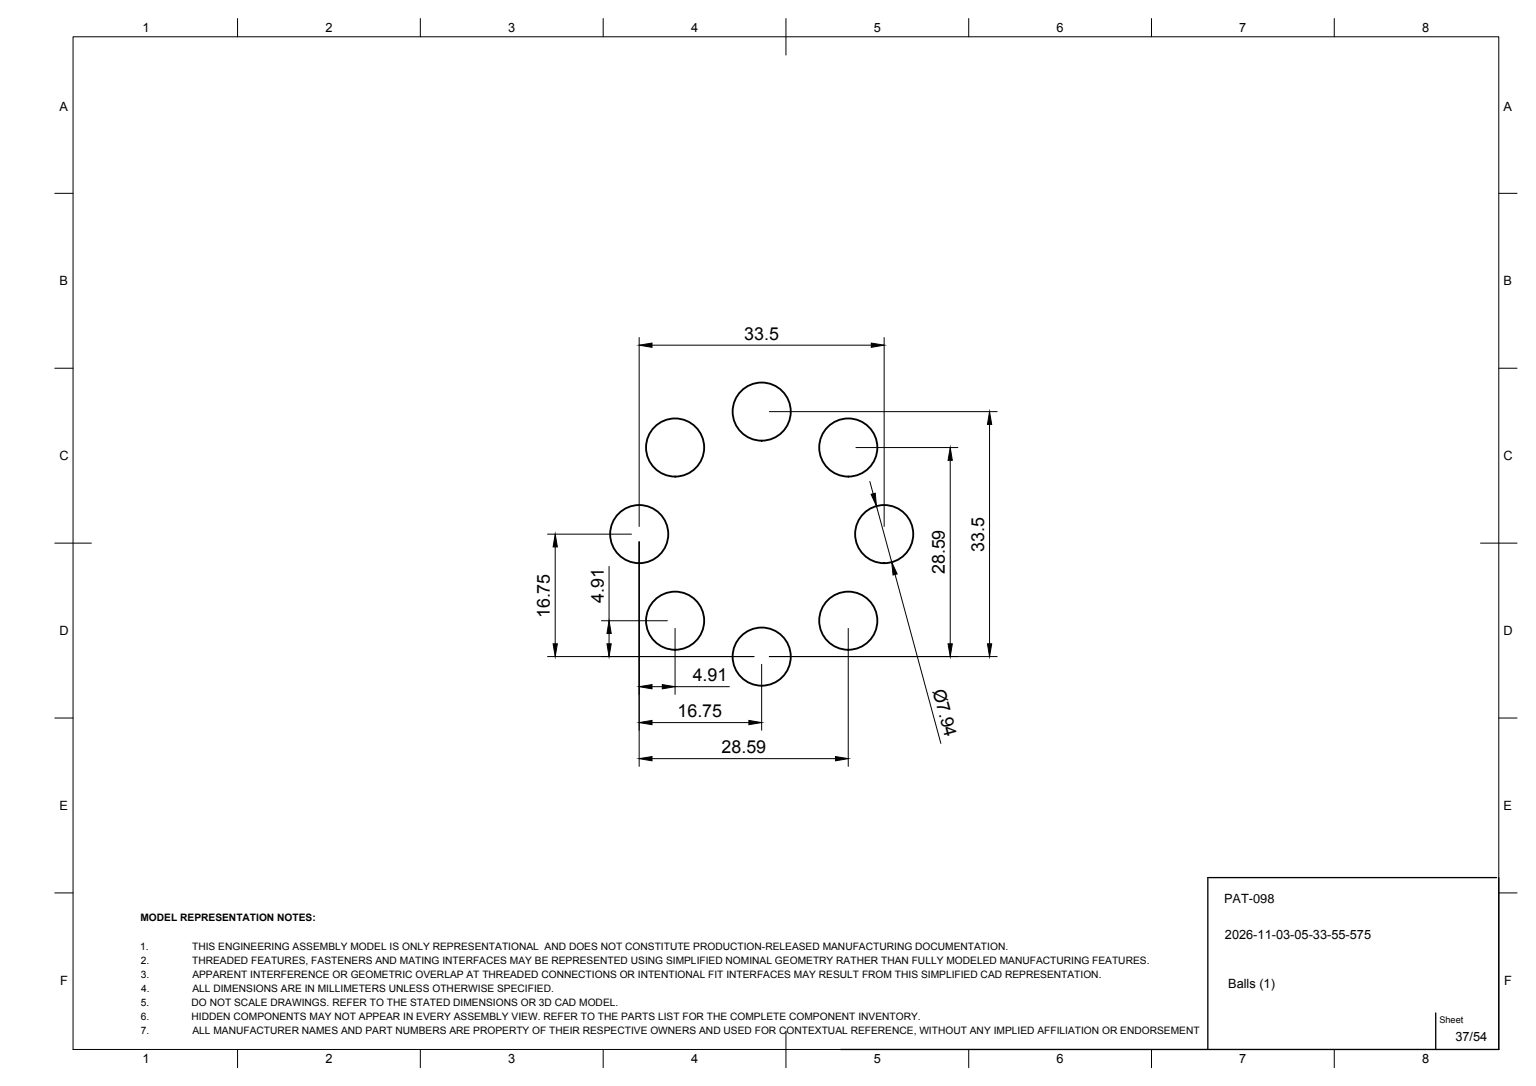
ISO-10303-21;
HEADER;
/* Generated by software containing ST-Developer
 * from STEP Tools, Inc. (www.steptools.com) 
 */

FILE_DESCRIPTION(
/* description */ ('Spring compression tester'),
/* implementation_level */ '2;1');

FILE_NAME(
/* name */ 'Balls (1).step',
/* time_stamp */ '2026-10-28T03:24:11-07:00',
/* author */ (''),
/* organization */ (''),
/* preprocessor_version */ 'ST-DEVELOPER v20.2',
/* originating_system */ 'Autodesk Translation Framework v15.17.0.0',
/* authorisation */ '');

FILE_SCHEMA (('AUTOMOTIVE_DESIGN { 1 0 10303 214 3 1 1 }'));
ENDSEC;

DATA;
#10=MECHANICAL_DESIGN_GEOMETRIC_PRESENTATION_REPRESENTATION('',(#1141,#1142,#1143,#1144,#1145,#1146,#1147,#1148),#43521);
#911=SPHERICAL_SURFACE('',#20162,0.3969);
#912=SPHERICAL_SURFACE('',#20164,0.3969);
#913=SPHERICAL_SURFACE('',#20166,0.3969);
#914=SPHERICAL_SURFACE('',#20168,0.3969);
#915=SPHERICAL_SURFACE('',#20170,0.3969);
#916=SPHERICAL_SURFACE('',#20172,0.3969);
#917=SPHERICAL_SURFACE('',#20174,0.3969);
#918=SPHERICAL_SURFACE('',#20176,0.3969);
#1014=SHAPE_REPRESENTATION_RELATIONSHIP('SRR','None',#43828,#1074);
#1074=ADVANCED_BREP_SHAPE_REPRESENTATION('',(#1215,#1216,#1217,#1218,#1219,
#1220,#1221,#1222),#43488);
#1141=STYLED_ITEM('',(#44202),#1215);
#1142=STYLED_ITEM('',(#44202),#1216);
#1143=STYLED_ITEM('',(#44202),#1217);
#1144=STYLED_ITEM('',(#44202),#1218);
#1145=STYLED_ITEM('',(#44202),#1219);
#1146=STYLED_ITEM('',(#44202),#1220);
#1147=STYLED_ITEM('',(#44202),#1221);
#1148=STYLED_ITEM('',(#44202),#1222);
#1215=MANIFOLD_SOLID_BREP('Body1',#18579);
#1216=MANIFOLD_SOLID_BREP('Body2',#18580);
#1217=MANIFOLD_SOLID_BREP('Body3',#18581);
#1218=MANIFOLD_SOLID_BREP('Body4',#18582);
#1219=MANIFOLD_SOLID_BREP('Body5',#18583);
#1220=MANIFOLD_SOLID_BREP('Body6',#18584);
#1221=MANIFOLD_SOLID_BREP('Body7',#18585);
#1222=MANIFOLD_SOLID_BREP('Body8',#18586);
#2660=FACE_OUTER_BOUND('',#3923,.T.);
#2661=FACE_OUTER_BOUND('',#3924,.T.);
#2662=FACE_OUTER_BOUND('',#3925,.T.);
#2663=FACE_OUTER_BOUND('',#3926,.T.);
#2664=FACE_OUTER_BOUND('',#3927,.T.);
#2665=FACE_OUTER_BOUND('',#3928,.T.);
#2666=FACE_OUTER_BOUND('',#3929,.T.);
#2667=FACE_OUTER_BOUND('',#3930,.T.);
#3923=EDGE_LOOP('',(#14383,#14384));
#3924=EDGE_LOOP('',(#14385,#14386));
#3925=EDGE_LOOP('',(#14387,#14388));
#3926=EDGE_LOOP('',(#14389,#14390));
#3927=EDGE_LOOP('',(#14391,#14392));
#3928=EDGE_LOOP('',(#14393,#14394));
#3929=EDGE_LOOP('',(#14395,#14396));
#3930=EDGE_LOOP('',(#14397,#14398));
#7818=CIRCLE('',#20163,0.3969);
#7819=CIRCLE('',#20165,0.3969);
#7820=CIRCLE('',#20167,0.3969);
#7821=CIRCLE('',#20169,0.3969);
#7822=CIRCLE('',#20171,0.3969);
#7823=CIRCLE('',#20173,0.3969);
#7824=CIRCLE('',#20175,0.3969);
#7825=CIRCLE('',#20177,0.3969);
#8863=VERTEX_POINT('',#29087);
#8864=VERTEX_POINT('',#29088);
#8865=VERTEX_POINT('',#29091);
#8866=VERTEX_POINT('',#29092);
#8867=VERTEX_POINT('',#29095);
#8868=VERTEX_POINT('',#29096);
#8869=VERTEX_POINT('',#29099);
#8870=VERTEX_POINT('',#29100);
#8871=VERTEX_POINT('',#29103);
#8872=VERTEX_POINT('',#29104);
#8873=VERTEX_POINT('',#29107);
#8874=VERTEX_POINT('',#29108);
#8875=VERTEX_POINT('',#29111);
#8876=VERTEX_POINT('',#29112);
#8877=VERTEX_POINT('',#29115);
#8878=VERTEX_POINT('',#29116);
#10856=EDGE_CURVE('',#8863,#8864,#7818,.T.);
#10857=EDGE_CURVE('',#8865,#8866,#7819,.T.);
#10858=EDGE_CURVE('',#8867,#8868,#7820,.T.);
#10859=EDGE_CURVE('',#8869,#8870,#7821,.T.);
#10860=EDGE_CURVE('',#8871,#8872,#7822,.T.);
#10861=EDGE_CURVE('',#8873,#8874,#7823,.T.);
#10862=EDGE_CURVE('',#8875,#8876,#7824,.T.);
#10863=EDGE_CURVE('',#8877,#8878,#7825,.T.);
#14383=ORIENTED_EDGE('',*,*,#10856,.T.);
#14384=ORIENTED_EDGE('',*,*,#10856,.F.);
#14385=ORIENTED_EDGE('',*,*,#10857,.T.);
#14386=ORIENTED_EDGE('',*,*,#10857,.F.);
#14387=ORIENTED_EDGE('',*,*,#10858,.T.);
#14388=ORIENTED_EDGE('',*,*,#10858,.F.);
#14389=ORIENTED_EDGE('',*,*,#10859,.T.);
#14390=ORIENTED_EDGE('',*,*,#10859,.F.);
#14391=ORIENTED_EDGE('',*,*,#10860,.T.);
#14392=ORIENTED_EDGE('',*,*,#10860,.F.);
#14393=ORIENTED_EDGE('',*,*,#10861,.T.);
#14394=ORIENTED_EDGE('',*,*,#10861,.F.);
#14395=ORIENTED_EDGE('',*,*,#10862,.T.);
#14396=ORIENTED_EDGE('',*,*,#10862,.F.);
#14397=ORIENTED_EDGE('',*,*,#10863,.T.);
#14398=ORIENTED_EDGE('',*,*,#10863,.F.);
#17984=ADVANCED_FACE('',(#2660),#911,.T.);
#17985=ADVANCED_FACE('',(#2661),#912,.T.);
#17986=ADVANCED_FACE('',(#2662),#913,.T.);
#17987=ADVANCED_FACE('',(#2663),#914,.T.);
#17988=ADVANCED_FACE('',(#2664),#915,.T.);
#17989=ADVANCED_FACE('',(#2665),#916,.T.);
#17990=ADVANCED_FACE('',(#2666),#917,.T.);
#17991=ADVANCED_FACE('',(#2667),#918,.T.);
#18579=CLOSED_SHELL('',(#17984));
#18580=CLOSED_SHELL('',(#17985));
#18581=CLOSED_SHELL('',(#17986));
#18582=CLOSED_SHELL('',(#17987));
#18583=CLOSED_SHELL('',(#17988));
#18584=CLOSED_SHELL('',(#17989));
#18585=CLOSED_SHELL('',(#17990));
#18586=CLOSED_SHELL('',(#17991));
#20161=AXIS2_PLACEMENT_3D('',#29085,#23671,#23672);
#20162=AXIS2_PLACEMENT_3D('',#29086,#23673,#23674);
#20163=AXIS2_PLACEMENT_3D('',#29089,#23675,#23676);
#20164=AXIS2_PLACEMENT_3D('',#29090,#23677,#23678);
#20165=AXIS2_PLACEMENT_3D('',#29093,#23679,#23680);
#20166=AXIS2_PLACEMENT_3D('',#29094,#23681,#23682);
#20167=AXIS2_PLACEMENT_3D('',#29097,#23683,#23684);
#20168=AXIS2_PLACEMENT_3D('',#29098,#23685,#23686);
#20169=AXIS2_PLACEMENT_3D('',#29101,#23687,#23688);
#20170=AXIS2_PLACEMENT_3D('',#29102,#23689,#23690);
#20171=AXIS2_PLACEMENT_3D('',#29105,#23691,#23692);
#20172=AXIS2_PLACEMENT_3D('',#29106,#23693,#23694);
#20173=AXIS2_PLACEMENT_3D('',#29109,#23695,#23696);
#20174=AXIS2_PLACEMENT_3D('',#29110,#23697,#23698);
#20175=AXIS2_PLACEMENT_3D('',#29113,#23699,#23700);
#20176=AXIS2_PLACEMENT_3D('',#29114,#23701,#23702);
#20177=AXIS2_PLACEMENT_3D('',#29117,#23703,#23704);
#23671=DIRECTION('axis',(0.,0.,1.));
#23672=DIRECTION('refdir',(1.,0.,0.));
#23673=DIRECTION('center_axis',(0.,0.,1.));
#23674=DIRECTION('ref_axis',(1.,0.,0.));
#23675=DIRECTION('center_axis',(1.22464679914735E-16,-1.,0.));
#23676=DIRECTION('ref_axis',(-1.,-1.22464679914735E-16,0.));
#23677=DIRECTION('center_axis',(0.707106781186548,0.,0.707106781186548));
#23678=DIRECTION('ref_axis',(0.707106781186548,0.,-0.707106781186548));
#23679=DIRECTION('center_axis',(8.65956056235493E-17,-1.,-8.65956056235493E-17));
#23680=DIRECTION('ref_axis',(-0.707106781186548,-1.22464679914735E-16,0.707106781186548));
#23681=DIRECTION('center_axis',(1.,0.,0.));
#23682=DIRECTION('ref_axis',(6.12323399573677E-17,0.,-1.));
#23683=DIRECTION('center_axis',(7.49879891330929E-33,-1.,-1.22464679914735E-16));
#23684=DIRECTION('ref_axis',(-6.12323399573677E-17,-1.22464679914735E-16,
1.));
#23685=DIRECTION('center_axis',(0.707106781186548,0.,-0.707106781186548));
#23686=DIRECTION('ref_axis',(-0.707106781186548,0.,-0.707106781186548));
#23687=DIRECTION('center_axis',(-8.65956056235493E-17,-1.,-8.65956056235493E-17));
#23688=DIRECTION('ref_axis',(0.707106781186548,-1.22464679914735E-16,0.707106781186548));
#23689=DIRECTION('center_axis',(0.,0.,-1.));
#23690=DIRECTION('ref_axis',(-1.,0.,-1.22464679914735E-16));
#23691=DIRECTION('center_axis',(-1.22464679914735E-16,-1.,-1.49975978266186E-32));
#23692=DIRECTION('ref_axis',(1.,-1.22464679914735E-16,1.22464679914735E-16));
#23693=DIRECTION('center_axis',(-0.707106781186548,0.,-0.707106781186548));
#23694=DIRECTION('ref_axis',(-0.707106781186548,0.,0.707106781186548));
#23695=DIRECTION('center_axis',(-8.65956056235493E-17,-1.,8.65956056235493E-17));
#23696=DIRECTION('ref_axis',(0.707106781186548,-1.22464679914735E-16,-0.707106781186548));
#23697=DIRECTION('center_axis',(-1.,0.,0.));
#23698=DIRECTION('ref_axis',(-1.83697019872103E-16,0.,1.));
#23699=DIRECTION('center_axis',(-2.24963967399279E-32,-1.,1.22464679914735E-16));
#23700=DIRECTION('ref_axis',(1.83697019872103E-16,-1.22464679914735E-16,
-1.));
#23701=DIRECTION('center_axis',(-0.707106781186548,0.,0.707106781186548));
#23702=DIRECTION('ref_axis',(0.707106781186548,0.,0.707106781186548));
#23703=DIRECTION('center_axis',(8.65956056235493E-17,-1.,8.65956056235494E-17));
#23704=DIRECTION('ref_axis',(-0.707106781186548,-1.22464679914735E-16,-0.707106781186548));
#29085=CARTESIAN_POINT('',(0.,0.,0.));
#29086=CARTESIAN_POINT('Origin',(1.675,0.,0.));
#29087=CARTESIAN_POINT('',(1.675,-2.97627328869245E-33,0.3969));
#29088=CARTESIAN_POINT('',(1.675,-2.97627328869245E-33,-0.3969));
#29089=CARTESIAN_POINT('Origin',(1.675,0.,0.));
#29090=CARTESIAN_POINT('Origin',(1.18440385848747,0.,-1.18440385848747));
#29091=CARTESIAN_POINT('',(1.46505453994041,3.1867025333467E-33,-0.903753177034526));
#29092=CARTESIAN_POINT('',(0.903753177034527,-9.13924911073161E-33,-1.46505453994041));
#29093=CARTESIAN_POINT('Origin',(1.18440385848747,0.,-1.18440385848747));
#29094=CARTESIAN_POINT('Origin',(1.02564169428591E-16,0.,-1.675));
#29095=CARTESIAN_POINT('',(0.3969,-2.97627328869246E-33,-1.675));
#29096=CARTESIAN_POINT('',(-0.3969,-2.97627328869245E-33,-1.675));
#29097=CARTESIAN_POINT('Origin',(1.02564169428591E-16,0.,-1.675));
#29098=CARTESIAN_POINT('Origin',(-1.18440385848747,0.,-1.18440385848747));
#29099=CARTESIAN_POINT('',(-0.903753177034526,3.1867025333467E-33,-1.46505453994041));
#29100=CARTESIAN_POINT('',(-1.46505453994041,-9.13924911073161E-33,-0.903753177034527));
#29101=CARTESIAN_POINT('Origin',(-1.18440385848747,0.,-1.18440385848747));
#29102=CARTESIAN_POINT('Origin',(-1.675,0.,-2.05128338857182E-16));
#29103=CARTESIAN_POINT('',(-1.675,-2.97627328869246E-33,-0.3969));
#29104=CARTESIAN_POINT('',(-1.675,-2.97627328869245E-33,0.3969));
#29105=CARTESIAN_POINT('Origin',(-1.675,0.,-2.05128338857182E-16));
#29106=CARTESIAN_POINT('Origin',(-1.18440385848747,0.,1.18440385848747));
#29107=CARTESIAN_POINT('',(-1.46505453994041,6.26819044436628E-33,0.903753177034526));
#29108=CARTESIAN_POINT('',(-0.903753177034527,-1.22207370217512E-32,1.46505453994041));
#29109=CARTESIAN_POINT('Origin',(-1.18440385848747,0.,1.18440385848747));
#29110=CARTESIAN_POINT('Origin',(-3.07692508285772E-16,0.,1.675));
#29111=CARTESIAN_POINT('',(-0.3969,-2.97627328869246E-33,1.675));
#29112=CARTESIAN_POINT('',(0.396899999999999,-2.97627328869245E-33,1.675));
#29113=CARTESIAN_POINT('Origin',(-3.07692508285772E-16,0.,1.675));
#29114=CARTESIAN_POINT('Origin',(1.18440385848747,0.,1.18440385848747));
#29115=CARTESIAN_POINT('',(0.903753177034526,9.34967835538585E-33,1.46505453994041));
#29116=CARTESIAN_POINT('',(1.46505453994041,-1.53022249327708E-32,0.903753177034527));
#29117=CARTESIAN_POINT('Origin',(1.18440385848747,0.,1.18440385848747));
#43420=UNCERTAINTY_MEASURE_WITH_UNIT(LENGTH_MEASURE(0.001),#43522,
'DISTANCE_ACCURACY_VALUE',
'Maximum model space distance between geometric entities at asserted c
onnectivities');
#43453=UNCERTAINTY_MEASURE_WITH_UNIT(LENGTH_MEASURE(0.001),#43522,
'DISTANCE_ACCURACY_VALUE',
'Maximum model space distance between geometric entities at asserted c
onnectivities');
#43488=(
GEOMETRIC_REPRESENTATION_CONTEXT(3)
GLOBAL_UNCERTAINTY_ASSIGNED_CONTEXT((#43420))
GLOBAL_UNIT_ASSIGNED_CONTEXT((#43522,#43524,#43525))
REPRESENTATION_CONTEXT('','3D')
);
#43521=(
GEOMETRIC_REPRESENTATION_CONTEXT(3)
GLOBAL_UNCERTAINTY_ASSIGNED_CONTEXT((#43453))
GLOBAL_UNIT_ASSIGNED_CONTEXT((#43522,#43524,#43525))
REPRESENTATION_CONTEXT('','3D')
);
#43522=(
LENGTH_UNIT()
NAMED_UNIT(*)
SI_UNIT(.CENTI.,.METRE.)
);
#43524=(
NAMED_UNIT(*)
PLANE_ANGLE_UNIT()
SI_UNIT($,.RADIAN.)
);
#43525=(
NAMED_UNIT(*)
SI_UNIT($,.STERADIAN.)
SOLID_ANGLE_UNIT()
);
#43560=SHAPE_DEFINITION_REPRESENTATION(#43632,#43828);
#43632=PRODUCT_DEFINITION_SHAPE('',$,#43896);
#43828=SHAPE_REPRESENTATION('',(#20161),#43488);
#43861=PRODUCT_DEFINITION_CONTEXT('part definition',#44064,'design');
#43896=PRODUCT_DEFINITION('Balls (1)','Balls (1)',#43963,#43861);
#43963=PRODUCT_DEFINITION_FORMATION('',$,#44100);
#44064=APPLICATION_CONTEXT(
'Core Data for Automotive Mechanical Design Process');
#44065=PRODUCT_CONTEXT('part definition',#44064,'mechanical');
#44100=PRODUCT('Balls (1)','Balls (1)','Balls (1)',(#44065));
#44196=COLOUR_RGB('Grey',0.48,0.52,0.57);
#44197=FILL_AREA_STYLE_COLOUR('',#44196);
#44198=FILL_AREA_STYLE('',(#44197));
#44199=SURFACE_STYLE_FILL_AREA(#44198);
#44200=SURFACE_SIDE_STYLE('',(#44199));
#44201=SURFACE_STYLE_USAGE(.BOTH.,#44200);
#44202=PRESENTATION_STYLE_ASSIGNMENT((#44201));
ENDSEC;
END-ISO-10303-21;
